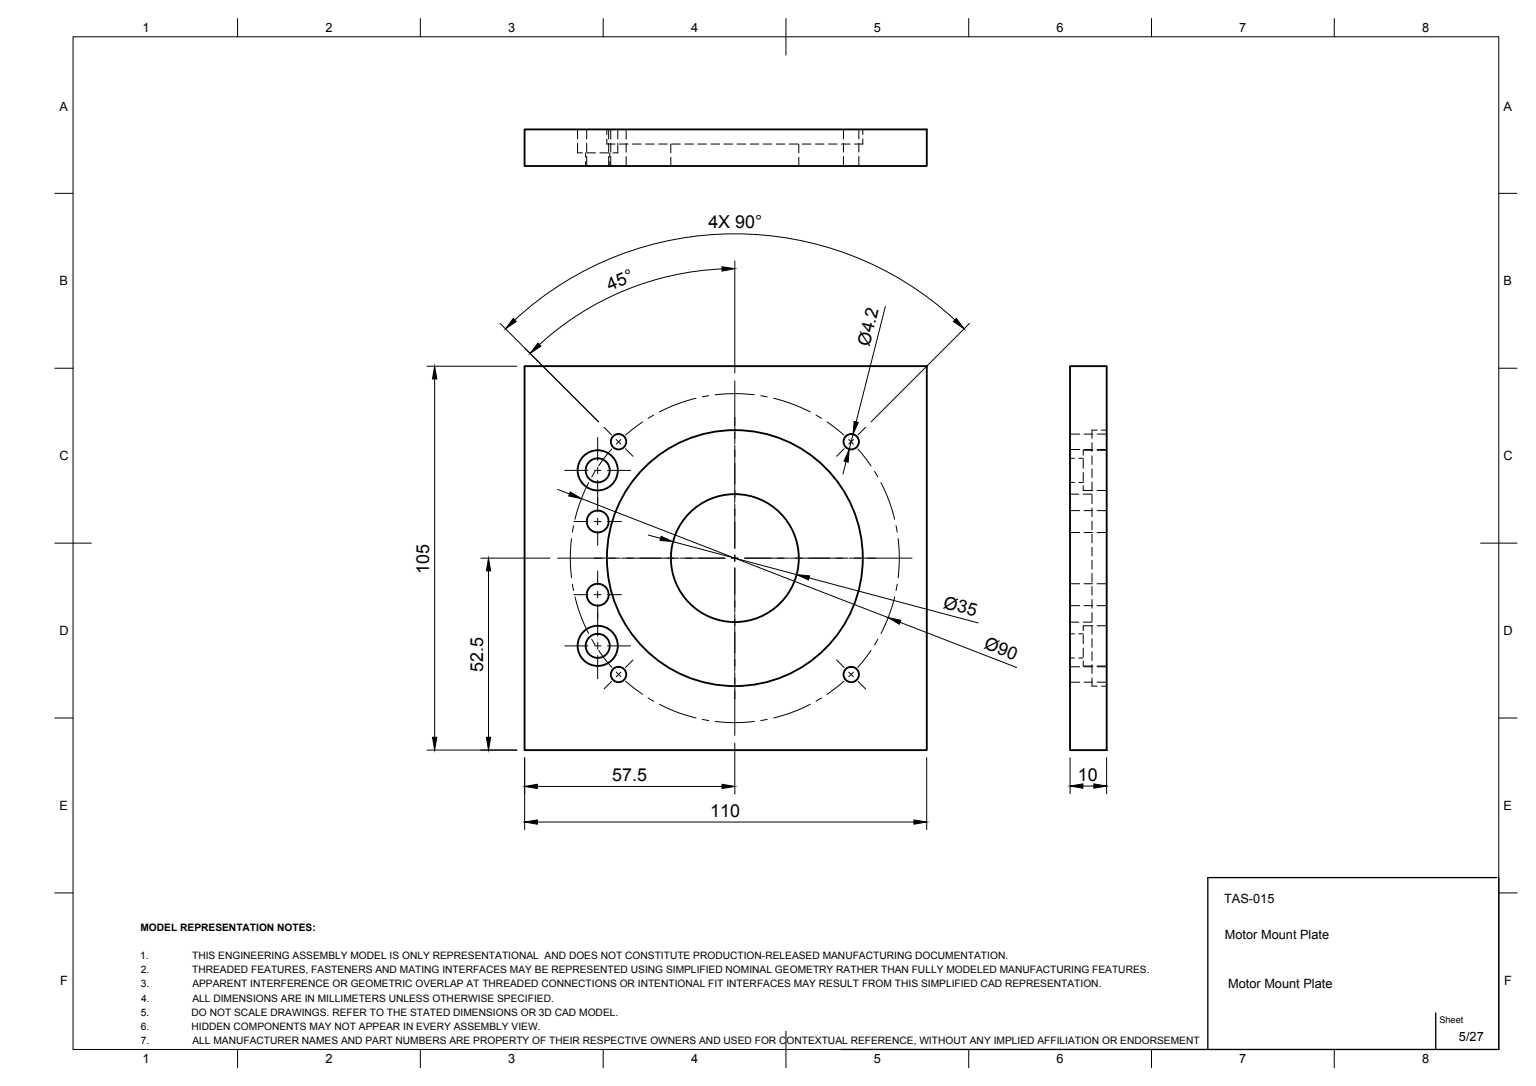
ISO-10303-21;
HEADER;
/* Generated by software containing ST-Developer
 * from STEP Tools, Inc. (www.steptools.com) 
 */

FILE_DESCRIPTION(
/* description */ ('STEP AP214'),
/* implementation_level */ '2;1');

FILE_NAME(
/* name */ 'Motor Mount Plate.step',
/* time_stamp */ '2026-11-15T14:49:54-08:00',
/* author */ (''),
/* organization */ (''),
/* preprocessor_version */ 'ST-DEVELOPER v20.2',
/* originating_system */ 'Autodesk Translation Framework v15.17.0.0',
/* authorisation */ '');

FILE_SCHEMA (('AUTOMOTIVE_DESIGN { 1 0 10303 214 3 1 1 }'));
ENDSEC;

DATA;
#10=MECHANICAL_DESIGN_GEOMETRIC_PRESENTATION_REPRESENTATION('',(#1100),#66721);
#1038=SHAPE_REPRESENTATION_RELATIONSHIP('SRR','None',#66894,#1069);
#1069=ADVANCED_BREP_SHAPE_REPRESENTATION('',(#1135),#66685);
#1100=STYLED_ITEM('',(#67095),#1135);
#1135=MANIFOLD_SOLID_BREP('Body1',#25666);
#1188=FACE_BOUND('',#3778,.T.);
#1189=FACE_BOUND('',#3779,.T.);
#1190=FACE_BOUND('',#3780,.T.);
#1191=FACE_BOUND('',#3781,.T.);
#1192=FACE_BOUND('',#3782,.T.);
#1193=FACE_BOUND('',#3783,.T.);
#1194=FACE_BOUND('',#3784,.T.);
#1195=FACE_BOUND('',#3785,.T.);
#1196=FACE_BOUND('',#3786,.T.);
#1197=FACE_BOUND('',#3792,.T.);
#1198=FACE_BOUND('',#3793,.T.);
#1199=FACE_BOUND('',#3794,.T.);
#1200=FACE_BOUND('',#3795,.T.);
#1201=FACE_BOUND('',#3796,.T.);
#1202=FACE_BOUND('',#3797,.T.);
#1203=FACE_BOUND('',#3798,.T.);
#1204=FACE_BOUND('',#3799,.T.);
#1205=FACE_BOUND('',#3800,.T.);
#1206=FACE_BOUND('',#3802,.T.);
#1207=FACE_BOUND('',#3804,.T.);
#1208=FACE_BOUND('',#3806,.T.);
#1524=PLANE('',#26132);
#1525=PLANE('',#26133);
#1526=PLANE('',#26134);
#1527=PLANE('',#26135);
#1528=PLANE('',#26136);
#1529=PLANE('',#26137);
#1530=PLANE('',#26138);
#1531=PLANE('',#26139);
#1532=PLANE('',#26140);
#2303=FACE_OUTER_BOUND('',#3765,.T.);
#2304=FACE_OUTER_BOUND('',#3766,.T.);
#2305=FACE_OUTER_BOUND('',#3767,.T.);
#2306=FACE_OUTER_BOUND('',#3768,.T.);
#2307=FACE_OUTER_BOUND('',#3769,.T.);
#2308=FACE_OUTER_BOUND('',#3770,.T.);
#2309=FACE_OUTER_BOUND('',#3771,.T.);
#2310=FACE_OUTER_BOUND('',#3772,.T.);
#2311=FACE_OUTER_BOUND('',#3773,.T.);
#2312=FACE_OUTER_BOUND('',#3774,.T.);
#2313=FACE_OUTER_BOUND('',#3775,.T.);
#2314=FACE_OUTER_BOUND('',#3776,.T.);
#2315=FACE_OUTER_BOUND('',#3777,.T.);
#2316=FACE_OUTER_BOUND('',#3787,.T.);
#2317=FACE_OUTER_BOUND('',#3788,.T.);
#2318=FACE_OUTER_BOUND('',#3789,.T.);
#2319=FACE_OUTER_BOUND('',#3790,.T.);
#2320=FACE_OUTER_BOUND('',#3791,.T.);
#2321=FACE_OUTER_BOUND('',#3801,.T.);
#2322=FACE_OUTER_BOUND('',#3803,.T.);
#2323=FACE_OUTER_BOUND('',#3805,.T.);
#3765=EDGE_LOOP('',(#16774,#16775,#16776,#16777));
#3766=EDGE_LOOP('',(#16778,#16779,#16780,#16781));
#3767=EDGE_LOOP('',(#16782,#16783,#16784,#16785));
#3768=EDGE_LOOP('',(#16786,#16787,#16788,#16789));
#3769=EDGE_LOOP('',(#16790,#16791,#16792,#16793));
#3770=EDGE_LOOP('',(#16794,#16795,#16796,#16797));
#3771=EDGE_LOOP('',(#16798,#16799,#16800,#16801));
#3772=EDGE_LOOP('',(#16802,#16803,#16804,#16805));
#3773=EDGE_LOOP('',(#16806,#16807,#16808,#16809));
#3774=EDGE_LOOP('',(#16810,#16811,#16812,#16813));
#3775=EDGE_LOOP('',(#16814,#16815,#16816,#16817));
#3776=EDGE_LOOP('',(#16818,#16819,#16820,#16821));
#3777=EDGE_LOOP('',(#16822,#16823,#16824,#16825));
#3778=EDGE_LOOP('',(#16826));
#3779=EDGE_LOOP('',(#16827));
#3780=EDGE_LOOP('',(#16828));
#3781=EDGE_LOOP('',(#16829));
#3782=EDGE_LOOP('',(#16830));
#3783=EDGE_LOOP('',(#16831));
#3784=EDGE_LOOP('',(#16832));
#3785=EDGE_LOOP('',(#16833));
#3786=EDGE_LOOP('',(#16834));
#3787=EDGE_LOOP('',(#16835,#16836,#16837,#16838));
#3788=EDGE_LOOP('',(#16839,#16840,#16841,#16842));
#3789=EDGE_LOOP('',(#16843,#16844,#16845,#16846));
#3790=EDGE_LOOP('',(#16847,#16848,#16849,#16850));
#3791=EDGE_LOOP('',(#16851,#16852,#16853,#16854));
#3792=EDGE_LOOP('',(#16855));
#3793=EDGE_LOOP('',(#16856));
#3794=EDGE_LOOP('',(#16857));
#3795=EDGE_LOOP('',(#16858));
#3796=EDGE_LOOP('',(#16859));
#3797=EDGE_LOOP('',(#16860));
#3798=EDGE_LOOP('',(#16861));
#3799=EDGE_LOOP('',(#16862));
#3800=EDGE_LOOP('',(#16863));
#3801=EDGE_LOOP('',(#16864));
#3802=EDGE_LOOP('',(#16865));
#3803=EDGE_LOOP('',(#16866));
#3804=EDGE_LOOP('',(#16867));
#3805=EDGE_LOOP('',(#16868));
#3806=EDGE_LOOP('',(#16869));
#5557=LINE('',#36368,#7546);
#5558=LINE('',#36374,#7547);
#5559=LINE('',#36380,#7548);
#5560=LINE('',#36386,#7549);
#5561=LINE('',#36392,#7550);
#5562=LINE('',#36398,#7551);
#5563=LINE('',#36404,#7552);
#5564=LINE('',#36410,#7553);
#5565=LINE('',#36416,#7554);
#5566=LINE('',#36422,#7555);
#5567=LINE('',#36428,#7556);
#5568=LINE('',#36434,#7557);
#5569=LINE('',#36439,#7558);
#5570=LINE('',#36441,#7559);
#5571=LINE('',#36443,#7560);
#5572=LINE('',#36444,#7561);
#5573=LINE('',#36447,#7562);
#5574=LINE('',#36449,#7563);
#5575=LINE('',#36450,#7564);
#5576=LINE('',#36453,#7565);
#5577=LINE('',#36454,#7566);
#5578=LINE('',#36457,#7567);
#5579=LINE('',#36458,#7568);
#5580=LINE('',#36460,#7569);
#7546=VECTOR('',#28944,2.1);
#7547=VECTOR('',#28951,2.1);
#7548=VECTOR('',#28958,2.1);
#7549=VECTOR('',#28965,2.1);
#7550=VECTOR('',#28972,3.);
#7551=VECTOR('',#28979,3.);
#7552=VECTOR('',#28986,5.5);
#7553=VECTOR('',#28993,3.3);
#7554=VECTOR('',#29000,5.5);
#7555=VECTOR('',#29007,3.3);
#7556=VECTOR('',#29014,17.5);
#7557=VECTOR('',#29021,35.);
#7558=VECTOR('',#29026,1000.);
#7559=VECTOR('',#29027,1000.);
#7560=VECTOR('',#29028,1000.);
#7561=VECTOR('',#29029,1000.);
#7562=VECTOR('',#29032,1000.);
#7563=VECTOR('',#29033,1000.);
#7564=VECTOR('',#29034,1000.);
#7565=VECTOR('',#29037,1000.);
#7566=VECTOR('',#29038,1000.);
#7567=VECTOR('',#29041,1000.);
#7568=VECTOR('',#29042,1000.);
#7569=VECTOR('',#29045,1000.);
#9477=CIRCLE('',#26097,2.1);
#9478=CIRCLE('',#26098,2.1);
#9479=CIRCLE('',#26100,2.1);
#9480=CIRCLE('',#26101,2.1);
#9481=CIRCLE('',#26103,2.1);
#9482=CIRCLE('',#26104,2.1);
#9483=CIRCLE('',#26106,2.1);
#9484=CIRCLE('',#26107,2.1);
#9485=CIRCLE('',#26109,3.);
#9486=CIRCLE('',#26110,3.);
#9487=CIRCLE('',#26112,3.);
#9488=CIRCLE('',#26113,3.);
#9489=CIRCLE('',#26115,5.5);
#9490=CIRCLE('',#26116,5.5);
#9491=CIRCLE('',#26118,3.3);
#9492=CIRCLE('',#26119,3.3);
#9493=CIRCLE('',#26121,5.5);
#9494=CIRCLE('',#26122,5.5);
#9495=CIRCLE('',#26124,3.3);
#9496=CIRCLE('',#26125,3.3);
#9497=CIRCLE('',#26127,17.5);
#9498=CIRCLE('',#26128,17.5);
#9499=CIRCLE('',#26130,35.);
#9500=CIRCLE('',#26131,35.);
#10698=VERTEX_POINT('',#36365);
#10699=VERTEX_POINT('',#36367);
#10700=VERTEX_POINT('',#36371);
#10701=VERTEX_POINT('',#36373);
#10702=VERTEX_POINT('',#36377);
#10703=VERTEX_POINT('',#36379);
#10704=VERTEX_POINT('',#36383);
#10705=VERTEX_POINT('',#36385);
#10706=VERTEX_POINT('',#36389);
#10707=VERTEX_POINT('',#36391);
#10708=VERTEX_POINT('',#36395);
#10709=VERTEX_POINT('',#36397);
#10710=VERTEX_POINT('',#36401);
#10711=VERTEX_POINT('',#36403);
#10712=VERTEX_POINT('',#36407);
#10713=VERTEX_POINT('',#36409);
#10714=VERTEX_POINT('',#36413);
#10715=VERTEX_POINT('',#36415);
#10716=VERTEX_POINT('',#36419);
#10717=VERTEX_POINT('',#36421);
#10718=VERTEX_POINT('',#36425);
#10719=VERTEX_POINT('',#36427);
#10720=VERTEX_POINT('',#36431);
#10721=VERTEX_POINT('',#36433);
#10722=VERTEX_POINT('',#36437);
#10723=VERTEX_POINT('',#36438);
#10724=VERTEX_POINT('',#36440);
#10725=VERTEX_POINT('',#36442);
#10726=VERTEX_POINT('',#36446);
#10727=VERTEX_POINT('',#36448);
#10728=VERTEX_POINT('',#36452);
#10729=VERTEX_POINT('',#36456);
#13080=EDGE_CURVE('',#10698,#10698,#9477,.T.);
#13081=EDGE_CURVE('',#10698,#10699,#5557,.T.);
#13082=EDGE_CURVE('',#10699,#10699,#9478,.T.);
#13083=EDGE_CURVE('',#10700,#10700,#9479,.T.);
#13084=EDGE_CURVE('',#10700,#10701,#5558,.T.);
#13085=EDGE_CURVE('',#10701,#10701,#9480,.T.);
#13086=EDGE_CURVE('',#10702,#10702,#9481,.T.);
#13087=EDGE_CURVE('',#10702,#10703,#5559,.T.);
#13088=EDGE_CURVE('',#10703,#10703,#9482,.T.);
#13089=EDGE_CURVE('',#10704,#10704,#9483,.T.);
#13090=EDGE_CURVE('',#10704,#10705,#5560,.T.);
#13091=EDGE_CURVE('',#10705,#10705,#9484,.T.);
#13092=EDGE_CURVE('',#10706,#10706,#9485,.T.);
#13093=EDGE_CURVE('',#10706,#10707,#5561,.T.);
#13094=EDGE_CURVE('',#10707,#10707,#9486,.T.);
#13095=EDGE_CURVE('',#10708,#10708,#9487,.T.);
#13096=EDGE_CURVE('',#10708,#10709,#5562,.T.);
#13097=EDGE_CURVE('',#10709,#10709,#9488,.T.);
#13098=EDGE_CURVE('',#10710,#10710,#9489,.T.);
#13099=EDGE_CURVE('',#10710,#10711,#5563,.T.);
#13100=EDGE_CURVE('',#10711,#10711,#9490,.T.);
#13101=EDGE_CURVE('',#10712,#10712,#9491,.T.);
#13102=EDGE_CURVE('',#10712,#10713,#5564,.T.);
#13103=EDGE_CURVE('',#10713,#10713,#9492,.T.);
#13104=EDGE_CURVE('',#10714,#10714,#9493,.T.);
#13105=EDGE_CURVE('',#10714,#10715,#5565,.T.);
#13106=EDGE_CURVE('',#10715,#10715,#9494,.T.);
#13107=EDGE_CURVE('',#10716,#10716,#9495,.T.);
#13108=EDGE_CURVE('',#10716,#10717,#5566,.T.);
#13109=EDGE_CURVE('',#10717,#10717,#9496,.T.);
#13110=EDGE_CURVE('',#10718,#10718,#9497,.T.);
#13111=EDGE_CURVE('',#10718,#10719,#5567,.T.);
#13112=EDGE_CURVE('',#10719,#10719,#9498,.T.);
#13113=EDGE_CURVE('',#10720,#10720,#9499,.T.);
#13114=EDGE_CURVE('',#10720,#10721,#5568,.T.);
#13115=EDGE_CURVE('',#10721,#10721,#9500,.T.);
#13116=EDGE_CURVE('',#10722,#10723,#5569,.T.);
#13117=EDGE_CURVE('',#10724,#10722,#5570,.T.);
#13118=EDGE_CURVE('',#10725,#10724,#5571,.T.);
#13119=EDGE_CURVE('',#10723,#10725,#5572,.T.);
#13120=EDGE_CURVE('',#10726,#10723,#5573,.T.);
#13121=EDGE_CURVE('',#10727,#10726,#5574,.T.);
#13122=EDGE_CURVE('',#10727,#10722,#5575,.T.);
#13123=EDGE_CURVE('',#10728,#10725,#5576,.T.);
#13124=EDGE_CURVE('',#10726,#10728,#5577,.T.);
#13125=EDGE_CURVE('',#10729,#10724,#5578,.T.);
#13126=EDGE_CURVE('',#10728,#10729,#5579,.T.);
#13127=EDGE_CURVE('',#10729,#10727,#5580,.T.);
#16774=ORIENTED_EDGE('',*,*,#13080,.F.);
#16775=ORIENTED_EDGE('',*,*,#13081,.T.);
#16776=ORIENTED_EDGE('',*,*,#13082,.T.);
#16777=ORIENTED_EDGE('',*,*,#13081,.F.);
#16778=ORIENTED_EDGE('',*,*,#13083,.F.);
#16779=ORIENTED_EDGE('',*,*,#13084,.T.);
#16780=ORIENTED_EDGE('',*,*,#13085,.T.);
#16781=ORIENTED_EDGE('',*,*,#13084,.F.);
#16782=ORIENTED_EDGE('',*,*,#13086,.F.);
#16783=ORIENTED_EDGE('',*,*,#13087,.T.);
#16784=ORIENTED_EDGE('',*,*,#13088,.T.);
#16785=ORIENTED_EDGE('',*,*,#13087,.F.);
#16786=ORIENTED_EDGE('',*,*,#13089,.F.);
#16787=ORIENTED_EDGE('',*,*,#13090,.T.);
#16788=ORIENTED_EDGE('',*,*,#13091,.T.);
#16789=ORIENTED_EDGE('',*,*,#13090,.F.);
#16790=ORIENTED_EDGE('',*,*,#13092,.F.);
#16791=ORIENTED_EDGE('',*,*,#13093,.T.);
#16792=ORIENTED_EDGE('',*,*,#13094,.T.);
#16793=ORIENTED_EDGE('',*,*,#13093,.F.);
#16794=ORIENTED_EDGE('',*,*,#13095,.F.);
#16795=ORIENTED_EDGE('',*,*,#13096,.T.);
#16796=ORIENTED_EDGE('',*,*,#13097,.T.);
#16797=ORIENTED_EDGE('',*,*,#13096,.F.);
#16798=ORIENTED_EDGE('',*,*,#13098,.F.);
#16799=ORIENTED_EDGE('',*,*,#13099,.T.);
#16800=ORIENTED_EDGE('',*,*,#13100,.T.);
#16801=ORIENTED_EDGE('',*,*,#13099,.F.);
#16802=ORIENTED_EDGE('',*,*,#13101,.F.);
#16803=ORIENTED_EDGE('',*,*,#13102,.T.);
#16804=ORIENTED_EDGE('',*,*,#13103,.T.);
#16805=ORIENTED_EDGE('',*,*,#13102,.F.);
#16806=ORIENTED_EDGE('',*,*,#13104,.F.);
#16807=ORIENTED_EDGE('',*,*,#13105,.T.);
#16808=ORIENTED_EDGE('',*,*,#13106,.T.);
#16809=ORIENTED_EDGE('',*,*,#13105,.F.);
#16810=ORIENTED_EDGE('',*,*,#13107,.F.);
#16811=ORIENTED_EDGE('',*,*,#13108,.T.);
#16812=ORIENTED_EDGE('',*,*,#13109,.T.);
#16813=ORIENTED_EDGE('',*,*,#13108,.F.);
#16814=ORIENTED_EDGE('',*,*,#13110,.F.);
#16815=ORIENTED_EDGE('',*,*,#13111,.T.);
#16816=ORIENTED_EDGE('',*,*,#13112,.T.);
#16817=ORIENTED_EDGE('',*,*,#13111,.F.);
#16818=ORIENTED_EDGE('',*,*,#13113,.F.);
#16819=ORIENTED_EDGE('',*,*,#13114,.T.);
#16820=ORIENTED_EDGE('',*,*,#13115,.T.);
#16821=ORIENTED_EDGE('',*,*,#13114,.F.);
#16822=ORIENTED_EDGE('',*,*,#13116,.F.);
#16823=ORIENTED_EDGE('',*,*,#13117,.F.);
#16824=ORIENTED_EDGE('',*,*,#13118,.F.);
#16825=ORIENTED_EDGE('',*,*,#13119,.F.);
#16826=ORIENTED_EDGE('',*,*,#13110,.T.);
#16827=ORIENTED_EDGE('',*,*,#13107,.T.);
#16828=ORIENTED_EDGE('',*,*,#13101,.T.);
#16829=ORIENTED_EDGE('',*,*,#13095,.T.);
#16830=ORIENTED_EDGE('',*,*,#13092,.T.);
#16831=ORIENTED_EDGE('',*,*,#13089,.T.);
#16832=ORIENTED_EDGE('',*,*,#13086,.T.);
#16833=ORIENTED_EDGE('',*,*,#13080,.T.);
#16834=ORIENTED_EDGE('',*,*,#13083,.T.);
#16835=ORIENTED_EDGE('',*,*,#13116,.T.);
#16836=ORIENTED_EDGE('',*,*,#13120,.F.);
#16837=ORIENTED_EDGE('',*,*,#13121,.F.);
#16838=ORIENTED_EDGE('',*,*,#13122,.T.);
#16839=ORIENTED_EDGE('',*,*,#13119,.T.);
#16840=ORIENTED_EDGE('',*,*,#13123,.F.);
#16841=ORIENTED_EDGE('',*,*,#13124,.F.);
#16842=ORIENTED_EDGE('',*,*,#13120,.T.);
#16843=ORIENTED_EDGE('',*,*,#13118,.T.);
#16844=ORIENTED_EDGE('',*,*,#13125,.F.);
#16845=ORIENTED_EDGE('',*,*,#13126,.F.);
#16846=ORIENTED_EDGE('',*,*,#13123,.T.);
#16847=ORIENTED_EDGE('',*,*,#13117,.T.);
#16848=ORIENTED_EDGE('',*,*,#13122,.F.);
#16849=ORIENTED_EDGE('',*,*,#13127,.F.);
#16850=ORIENTED_EDGE('',*,*,#13125,.T.);
#16851=ORIENTED_EDGE('',*,*,#13121,.T.);
#16852=ORIENTED_EDGE('',*,*,#13124,.T.);
#16853=ORIENTED_EDGE('',*,*,#13126,.T.);
#16854=ORIENTED_EDGE('',*,*,#13127,.T.);
#16855=ORIENTED_EDGE('',*,*,#13082,.F.);
#16856=ORIENTED_EDGE('',*,*,#13085,.F.);
#16857=ORIENTED_EDGE('',*,*,#13088,.F.);
#16858=ORIENTED_EDGE('',*,*,#13091,.F.);
#16859=ORIENTED_EDGE('',*,*,#13094,.F.);
#16860=ORIENTED_EDGE('',*,*,#13097,.F.);
#16861=ORIENTED_EDGE('',*,*,#13100,.F.);
#16862=ORIENTED_EDGE('',*,*,#13106,.F.);
#16863=ORIENTED_EDGE('',*,*,#13115,.F.);
#16864=ORIENTED_EDGE('',*,*,#13113,.T.);
#16865=ORIENTED_EDGE('',*,*,#13112,.F.);
#16866=ORIENTED_EDGE('',*,*,#13104,.T.);
#16867=ORIENTED_EDGE('',*,*,#13109,.F.);
#16868=ORIENTED_EDGE('',*,*,#13098,.T.);
#16869=ORIENTED_EDGE('',*,*,#13103,.F.);
#23810=CYLINDRICAL_SURFACE('',#26096,2.1);
#23811=CYLINDRICAL_SURFACE('',#26099,2.1);
#23812=CYLINDRICAL_SURFACE('',#26102,2.1);
#23813=CYLINDRICAL_SURFACE('',#26105,2.1);
#23814=CYLINDRICAL_SURFACE('',#26108,3.);
#23815=CYLINDRICAL_SURFACE('',#26111,3.);
#23816=CYLINDRICAL_SURFACE('',#26114,5.5);
#23817=CYLINDRICAL_SURFACE('',#26117,3.3);
#23818=CYLINDRICAL_SURFACE('',#26120,5.5);
#23819=CYLINDRICAL_SURFACE('',#26123,3.3);
#23820=CYLINDRICAL_SURFACE('',#26126,17.5);
#23821=CYLINDRICAL_SURFACE('',#26129,35.);
#24256=ADVANCED_FACE('',(#2303),#23810,.F.);
#24257=ADVANCED_FACE('',(#2304),#23811,.F.);
#24258=ADVANCED_FACE('',(#2305),#23812,.F.);
#24259=ADVANCED_FACE('',(#2306),#23813,.F.);
#24260=ADVANCED_FACE('',(#2307),#23814,.F.);
#24261=ADVANCED_FACE('',(#2308),#23815,.F.);
#24262=ADVANCED_FACE('',(#2309),#23816,.F.);
#24263=ADVANCED_FACE('',(#2310),#23817,.F.);
#24264=ADVANCED_FACE('',(#2311),#23818,.F.);
#24265=ADVANCED_FACE('',(#2312),#23819,.F.);
#24266=ADVANCED_FACE('',(#2313),#23820,.F.);
#24267=ADVANCED_FACE('',(#2314),#23821,.F.);
#24268=ADVANCED_FACE('',(#2315,#1188,#1189,#1190,#1191,#1192,#1193,#1194,
#1195,#1196),#1524,.T.);
#24269=ADVANCED_FACE('',(#2316),#1525,.F.);
#24270=ADVANCED_FACE('',(#2317),#1526,.F.);
#24271=ADVANCED_FACE('',(#2318),#1527,.F.);
#24272=ADVANCED_FACE('',(#2319),#1528,.F.);
#24273=ADVANCED_FACE('',(#2320,#1197,#1198,#1199,#1200,#1201,#1202,#1203,
#1204,#1205),#1529,.F.);
#24274=ADVANCED_FACE('',(#2321,#1206),#1530,.T.);
#24275=ADVANCED_FACE('',(#2322,#1207),#1531,.F.);
#24276=ADVANCED_FACE('',(#2323,#1208),#1532,.F.);
#25666=CLOSED_SHELL('',(#24256,#24257,#24258,#24259,#24260,#24261,#24262,
#24263,#24264,#24265,#24266,#24267,#24268,#24269,#24270,#24271,#24272,#24273,
#24274,#24275,#24276));
#26095=AXIS2_PLACEMENT_3D('',#36363,#28938,#28939);
#26096=AXIS2_PLACEMENT_3D('',#36364,#28940,#28941);
#26097=AXIS2_PLACEMENT_3D('',#36366,#28942,#28943);
#26098=AXIS2_PLACEMENT_3D('',#36369,#28945,#28946);
#26099=AXIS2_PLACEMENT_3D('',#36370,#28947,#28948);
#26100=AXIS2_PLACEMENT_3D('',#36372,#28949,#28950);
#26101=AXIS2_PLACEMENT_3D('',#36375,#28952,#28953);
#26102=AXIS2_PLACEMENT_3D('',#36376,#28954,#28955);
#26103=AXIS2_PLACEMENT_3D('',#36378,#28956,#28957);
#26104=AXIS2_PLACEMENT_3D('',#36381,#28959,#28960);
#26105=AXIS2_PLACEMENT_3D('',#36382,#28961,#28962);
#26106=AXIS2_PLACEMENT_3D('',#36384,#28963,#28964);
#26107=AXIS2_PLACEMENT_3D('',#36387,#28966,#28967);
#26108=AXIS2_PLACEMENT_3D('',#36388,#28968,#28969);
#26109=AXIS2_PLACEMENT_3D('',#36390,#28970,#28971);
#26110=AXIS2_PLACEMENT_3D('',#36393,#28973,#28974);
#26111=AXIS2_PLACEMENT_3D('',#36394,#28975,#28976);
#26112=AXIS2_PLACEMENT_3D('',#36396,#28977,#28978);
#26113=AXIS2_PLACEMENT_3D('',#36399,#28980,#28981);
#26114=AXIS2_PLACEMENT_3D('',#36400,#28982,#28983);
#26115=AXIS2_PLACEMENT_3D('',#36402,#28984,#28985);
#26116=AXIS2_PLACEMENT_3D('',#36405,#28987,#28988);
#26117=AXIS2_PLACEMENT_3D('',#36406,#28989,#28990);
#26118=AXIS2_PLACEMENT_3D('',#36408,#28991,#28992);
#26119=AXIS2_PLACEMENT_3D('',#36411,#28994,#28995);
#26120=AXIS2_PLACEMENT_3D('',#36412,#28996,#28997);
#26121=AXIS2_PLACEMENT_3D('',#36414,#28998,#28999);
#26122=AXIS2_PLACEMENT_3D('',#36417,#29001,#29002);
#26123=AXIS2_PLACEMENT_3D('',#36418,#29003,#29004);
#26124=AXIS2_PLACEMENT_3D('',#36420,#29005,#29006);
#26125=AXIS2_PLACEMENT_3D('',#36423,#29008,#29009);
#26126=AXIS2_PLACEMENT_3D('',#36424,#29010,#29011);
#26127=AXIS2_PLACEMENT_3D('',#36426,#29012,#29013);
#26128=AXIS2_PLACEMENT_3D('',#36429,#29015,#29016);
#26129=AXIS2_PLACEMENT_3D('',#36430,#29017,#29018);
#26130=AXIS2_PLACEMENT_3D('',#36432,#29019,#29020);
#26131=AXIS2_PLACEMENT_3D('',#36435,#29022,#29023);
#26132=AXIS2_PLACEMENT_3D('',#36436,#29024,#29025);
#26133=AXIS2_PLACEMENT_3D('',#36445,#29030,#29031);
#26134=AXIS2_PLACEMENT_3D('',#36451,#29035,#29036);
#26135=AXIS2_PLACEMENT_3D('',#36455,#29039,#29040);
#26136=AXIS2_PLACEMENT_3D('',#36459,#29043,#29044);
#26137=AXIS2_PLACEMENT_3D('',#36461,#29046,#29047);
#26138=AXIS2_PLACEMENT_3D('',#36462,#29048,#29049);
#26139=AXIS2_PLACEMENT_3D('',#36463,#29050,#29051);
#26140=AXIS2_PLACEMENT_3D('',#36464,#29052,#29053);
#28938=DIRECTION('axis',(0.,0.,1.));
#28939=DIRECTION('refdir',(1.,0.,0.));
#28940=DIRECTION('center_axis',(0.,0.,1.));
#28941=DIRECTION('ref_axis',(1.,0.,0.));
#28942=DIRECTION('center_axis',(0.,0.,1.));
#28943=DIRECTION('ref_axis',(1.,0.,0.));
#28944=DIRECTION('',(0.,0.,1.));
#28945=DIRECTION('center_axis',(0.,0.,1.));
#28946=DIRECTION('ref_axis',(1.,0.,0.));
#28947=DIRECTION('center_axis',(0.,0.,1.));
#28948=DIRECTION('ref_axis',(1.,0.,0.));
#28949=DIRECTION('center_axis',(0.,0.,1.));
#28950=DIRECTION('ref_axis',(1.,0.,0.));
#28951=DIRECTION('',(0.,0.,1.));
#28952=DIRECTION('center_axis',(0.,0.,1.));
#28953=DIRECTION('ref_axis',(1.,0.,0.));
#28954=DIRECTION('center_axis',(0.,0.,1.));
#28955=DIRECTION('ref_axis',(1.,0.,0.));
#28956=DIRECTION('center_axis',(0.,0.,1.));
#28957=DIRECTION('ref_axis',(1.,0.,0.));
#28958=DIRECTION('',(0.,0.,1.));
#28959=DIRECTION('center_axis',(0.,0.,1.));
#28960=DIRECTION('ref_axis',(1.,0.,0.));
#28961=DIRECTION('center_axis',(0.,0.,1.));
#28962=DIRECTION('ref_axis',(1.,0.,0.));
#28963=DIRECTION('center_axis',(0.,0.,1.));
#28964=DIRECTION('ref_axis',(1.,0.,0.));
#28965=DIRECTION('',(0.,0.,1.));
#28966=DIRECTION('center_axis',(0.,0.,1.));
#28967=DIRECTION('ref_axis',(1.,0.,0.));
#28968=DIRECTION('center_axis',(0.,0.,1.));
#28969=DIRECTION('ref_axis',(1.,0.,0.));
#28970=DIRECTION('center_axis',(0.,0.,1.));
#28971=DIRECTION('ref_axis',(1.,0.,0.));
#28972=DIRECTION('',(0.,0.,1.));
#28973=DIRECTION('center_axis',(0.,0.,1.));
#28974=DIRECTION('ref_axis',(1.,0.,0.));
#28975=DIRECTION('center_axis',(0.,0.,1.));
#28976=DIRECTION('ref_axis',(1.,0.,0.));
#28977=DIRECTION('center_axis',(0.,0.,1.));
#28978=DIRECTION('ref_axis',(1.,0.,0.));
#28979=DIRECTION('',(0.,0.,1.));
#28980=DIRECTION('center_axis',(0.,0.,1.));
#28981=DIRECTION('ref_axis',(1.,0.,0.));
#28982=DIRECTION('center_axis',(0.,0.,1.));
#28983=DIRECTION('ref_axis',(1.,0.,0.));
#28984=DIRECTION('center_axis',(0.,0.,1.));
#28985=DIRECTION('ref_axis',(1.,0.,0.));
#28986=DIRECTION('',(0.,0.,1.));
#28987=DIRECTION('center_axis',(0.,0.,1.));
#28988=DIRECTION('ref_axis',(1.,0.,0.));
#28989=DIRECTION('center_axis',(0.,0.,1.));
#28990=DIRECTION('ref_axis',(1.,0.,0.));
#28991=DIRECTION('center_axis',(0.,0.,1.));
#28992=DIRECTION('ref_axis',(1.,0.,0.));
#28993=DIRECTION('',(0.,0.,1.));
#28994=DIRECTION('center_axis',(0.,0.,1.));
#28995=DIRECTION('ref_axis',(1.,0.,0.));
#28996=DIRECTION('center_axis',(0.,0.,1.));
#28997=DIRECTION('ref_axis',(1.,0.,0.));
#28998=DIRECTION('center_axis',(0.,0.,1.));
#28999=DIRECTION('ref_axis',(1.,0.,0.));
#29000=DIRECTION('',(0.,0.,1.));
#29001=DIRECTION('center_axis',(0.,0.,1.));
#29002=DIRECTION('ref_axis',(1.,0.,0.));
#29003=DIRECTION('center_axis',(0.,0.,1.));
#29004=DIRECTION('ref_axis',(1.,0.,0.));
#29005=DIRECTION('center_axis',(0.,0.,1.));
#29006=DIRECTION('ref_axis',(1.,0.,0.));
#29007=DIRECTION('',(0.,0.,1.));
#29008=DIRECTION('center_axis',(0.,0.,1.));
#29009=DIRECTION('ref_axis',(1.,0.,0.));
#29010=DIRECTION('center_axis',(0.,0.,1.));
#29011=DIRECTION('ref_axis',(1.,0.,0.));
#29012=DIRECTION('center_axis',(0.,0.,1.));
#29013=DIRECTION('ref_axis',(1.,0.,0.));
#29014=DIRECTION('',(0.,0.,1.));
#29015=DIRECTION('center_axis',(0.,0.,1.));
#29016=DIRECTION('ref_axis',(1.,0.,0.));
#29017=DIRECTION('center_axis',(0.,0.,1.));
#29018=DIRECTION('ref_axis',(1.,0.,0.));
#29019=DIRECTION('center_axis',(0.,0.,1.));
#29020=DIRECTION('ref_axis',(1.,0.,0.));
#29021=DIRECTION('',(0.,0.,1.));
#29022=DIRECTION('center_axis',(0.,0.,1.));
#29023=DIRECTION('ref_axis',(1.,0.,0.));
#29024=DIRECTION('center_axis',(0.,0.,-1.));
#29025=DIRECTION('ref_axis',(-1.,0.,0.));
#29026=DIRECTION('',(0.,1.,0.));
#29027=DIRECTION('',(1.,0.,0.));
#29028=DIRECTION('',(0.,-1.,0.));
#29029=DIRECTION('',(-1.,0.,0.));
#29030=DIRECTION('center_axis',(-1.,0.,0.));
#29031=DIRECTION('ref_axis',(0.,0.,1.));
#29032=DIRECTION('',(0.,0.,-1.));
#29033=DIRECTION('',(0.,1.,0.));
#29034=DIRECTION('',(0.,0.,-1.));
#29035=DIRECTION('center_axis',(0.,-1.,0.));
#29036=DIRECTION('ref_axis',(0.,0.,-1.));
#29037=DIRECTION('',(0.,0.,-1.));
#29038=DIRECTION('',(-1.,0.,0.));
#29039=DIRECTION('center_axis',(1.,0.,0.));
#29040=DIRECTION('ref_axis',(0.,0.,-1.));
#29041=DIRECTION('',(0.,0.,-1.));
#29042=DIRECTION('',(0.,-1.,0.));
#29043=DIRECTION('center_axis',(0.,1.,0.));
#29044=DIRECTION('ref_axis',(0.,0.,1.));
#29045=DIRECTION('',(1.,0.,0.));
#29046=DIRECTION('center_axis',(0.,0.,-1.));
#29047=DIRECTION('ref_axis',(-1.,0.,0.));
#29048=DIRECTION('center_axis',(0.,0.,1.));
#29049=DIRECTION('ref_axis',(1.,0.,0.));
#29050=DIRECTION('center_axis',(0.,0.,-1.));
#29051=DIRECTION('ref_axis',(-1.,0.,0.));
#29052=DIRECTION('center_axis',(0.,0.,-1.));
#29053=DIRECTION('ref_axis',(-1.,0.,0.));
#36363=CARTESIAN_POINT('',(0.,0.,0.));
#36364=CARTESIAN_POINT('Origin',(31.819805153395,29.3198051533945,5.));
#36365=CARTESIAN_POINT('',(29.719805153395,29.3198051533945,-5.));
#36366=CARTESIAN_POINT('Origin',(31.819805153395,29.3198051533945,-5.));
#36367=CARTESIAN_POINT('',(29.719805153395,29.3198051533945,5.));
#36368=CARTESIAN_POINT('',(29.719805153395,29.3198051533945,5.));
#36369=CARTESIAN_POINT('Origin',(31.819805153395,29.3198051533945,5.));
#36370=CARTESIAN_POINT('Origin',(-31.8198051533946,29.319805153395,5.));
#36371=CARTESIAN_POINT('',(-33.9198051533946,29.319805153395,-5.));
#36372=CARTESIAN_POINT('Origin',(-31.8198051533946,29.319805153395,-5.));
#36373=CARTESIAN_POINT('',(-33.9198051533946,29.319805153395,5.));
#36374=CARTESIAN_POINT('',(-33.9198051533946,29.319805153395,5.));
#36375=CARTESIAN_POINT('Origin',(-31.8198051533946,29.319805153395,5.));
#36376=CARTESIAN_POINT('Origin',(-31.8198051533948,-34.3198051533942,5.));
#36377=CARTESIAN_POINT('',(-33.9198051533948,-34.3198051533942,-5.));
#36378=CARTESIAN_POINT('Origin',(-31.8198051533948,-34.3198051533942,-5.));
#36379=CARTESIAN_POINT('',(-33.9198051533948,-34.3198051533942,5.));
#36380=CARTESIAN_POINT('',(-33.9198051533948,-34.3198051533942,5.));
#36381=CARTESIAN_POINT('Origin',(-31.8198051533948,-34.3198051533942,5.));
#36382=CARTESIAN_POINT('Origin',(31.8198051533946,-34.3198051533944,5.));
#36383=CARTESIAN_POINT('',(29.7198051533946,-34.3198051533944,-5.));
#36384=CARTESIAN_POINT('Origin',(31.8198051533946,-34.3198051533944,-5.));
#36385=CARTESIAN_POINT('',(29.7198051533946,-34.3198051533944,5.));
#36386=CARTESIAN_POINT('',(29.7198051533946,-34.3198051533944,5.));
#36387=CARTESIAN_POINT('Origin',(31.8198051533946,-34.3198051533944,5.));
#36388=CARTESIAN_POINT('Origin',(-10.,35.,5.));
#36389=CARTESIAN_POINT('',(-13.,35.,-5.));
#36390=CARTESIAN_POINT('Origin',(-10.,35.,-5.));
#36391=CARTESIAN_POINT('',(-13.,35.,5.));
#36392=CARTESIAN_POINT('',(-13.,35.,5.));
#36393=CARTESIAN_POINT('Origin',(-10.,35.,5.));
#36394=CARTESIAN_POINT('Origin',(10.,35.,5.));
#36395=CARTESIAN_POINT('',(7.,35.,-5.));
#36396=CARTESIAN_POINT('Origin',(10.,35.,-5.));
#36397=CARTESIAN_POINT('',(7.,35.,5.));
#36398=CARTESIAN_POINT('',(7.,35.,5.));
#36399=CARTESIAN_POINT('Origin',(10.,35.,5.));
#36400=CARTESIAN_POINT('Origin',(-24.,35.,5.));
#36401=CARTESIAN_POINT('',(-29.5,35.,-1.4));
#36402=CARTESIAN_POINT('Origin',(-24.,35.,-1.4));
#36403=CARTESIAN_POINT('',(-29.5,35.,5.));
#36404=CARTESIAN_POINT('',(-29.5,35.,5.));
#36405=CARTESIAN_POINT('Origin',(-24.,35.,5.));
#36406=CARTESIAN_POINT('Origin',(-24.,35.,5.));
#36407=CARTESIAN_POINT('',(-27.3,35.,-5.));
#36408=CARTESIAN_POINT('Origin',(-24.,35.,-5.));
#36409=CARTESIAN_POINT('',(-27.3,35.,-1.4));
#36410=CARTESIAN_POINT('',(-27.3,35.,5.));
#36411=CARTESIAN_POINT('Origin',(-24.,35.,-1.4));
#36412=CARTESIAN_POINT('Origin',(24.,35.,5.));
#36413=CARTESIAN_POINT('',(18.5,35.,-1.4));
#36414=CARTESIAN_POINT('Origin',(24.,35.,-1.4));
#36415=CARTESIAN_POINT('',(18.5,35.,5.));
#36416=CARTESIAN_POINT('',(18.5,35.,5.));
#36417=CARTESIAN_POINT('Origin',(24.,35.,5.));
#36418=CARTESIAN_POINT('Origin',(24.,35.,5.));
#36419=CARTESIAN_POINT('',(20.7,35.,-5.));
#36420=CARTESIAN_POINT('Origin',(24.,35.,-5.));
#36421=CARTESIAN_POINT('',(20.7,35.,-1.4));
#36422=CARTESIAN_POINT('',(20.7,35.,5.));
#36423=CARTESIAN_POINT('Origin',(24.,35.,-1.4));
#36424=CARTESIAN_POINT('Origin',(-1.20882209737476E-14,-2.49999999999972,
-5.));
#36425=CARTESIAN_POINT('',(-17.5,-2.49999999999972,-5.));
#36426=CARTESIAN_POINT('Origin',(-1.20882209737476E-14,-2.49999999999972,
-5.));
#36427=CARTESIAN_POINT('',(-17.5,-2.49999999999972,1.));
#36428=CARTESIAN_POINT('',(-17.5,-2.49999999999972,-5.));
#36429=CARTESIAN_POINT('Origin',(-1.20882209737476E-14,-2.49999999999972,
1.));
#36430=CARTESIAN_POINT('Origin',(-1.20882209737476E-14,-2.49999999999972,
1.));
#36431=CARTESIAN_POINT('',(-35.,-2.49999999999972,1.));
#36432=CARTESIAN_POINT('Origin',(-1.20882209737476E-14,-2.49999999999972,
1.));
#36433=CARTESIAN_POINT('',(-35.,-2.49999999999972,5.));
#36434=CARTESIAN_POINT('',(-35.,-2.49999999999972,1.));
#36435=CARTESIAN_POINT('Origin',(-1.20882209737476E-14,-2.49999999999972,
5.));
#36436=CARTESIAN_POINT('Origin',(0.,0.,-5.));
#36437=CARTESIAN_POINT('',(52.5,-55.,-5.));
#36438=CARTESIAN_POINT('',(52.5,55.,-5.));
#36439=CARTESIAN_POINT('',(52.5,-55.,-5.));
#36440=CARTESIAN_POINT('',(-52.5,-55.,-5.));
#36441=CARTESIAN_POINT('',(-52.5,-55.,-5.));
#36442=CARTESIAN_POINT('',(-52.5,55.,-5.));
#36443=CARTESIAN_POINT('',(-52.5,-55.,-5.));
#36444=CARTESIAN_POINT('',(-52.5,55.,-5.));
#36445=CARTESIAN_POINT('Origin',(52.5,-55.,5.));
#36446=CARTESIAN_POINT('',(52.5,55.,5.));
#36447=CARTESIAN_POINT('',(52.5,55.,5.));
#36448=CARTESIAN_POINT('',(52.5,-55.,5.));
#36449=CARTESIAN_POINT('',(52.5,-55.,5.));
#36450=CARTESIAN_POINT('',(52.5,-55.,5.));
#36451=CARTESIAN_POINT('Origin',(-52.5,55.,5.));
#36452=CARTESIAN_POINT('',(-52.5,55.,5.));
#36453=CARTESIAN_POINT('',(-52.5,55.,5.));
#36454=CARTESIAN_POINT('',(-52.5,55.,5.));
#36455=CARTESIAN_POINT('Origin',(-52.5,-55.,5.));
#36456=CARTESIAN_POINT('',(-52.5,-55.,5.));
#36457=CARTESIAN_POINT('',(-52.5,-55.,5.));
#36458=CARTESIAN_POINT('',(-52.5,-55.,5.));
#36459=CARTESIAN_POINT('Origin',(-52.5,-55.,5.));
#36460=CARTESIAN_POINT('',(-52.5,-55.,5.));
#36461=CARTESIAN_POINT('Origin',(0.,0.,5.));
#36462=CARTESIAN_POINT('Origin',(-1.20882209737476E-14,-2.49999999999972,
1.));
#36463=CARTESIAN_POINT('Origin',(27.3,35.,-1.4));
#36464=CARTESIAN_POINT('Origin',(-20.7,35.,-1.4));
#66644=UNCERTAINTY_MEASURE_WITH_UNIT(LENGTH_MEASURE(0.01),#66722,
'DISTANCE_ACCURACY_VALUE',
'Maximum model space distance between geometric entities at asserted c
onnectivities');
#66680=UNCERTAINTY_MEASURE_WITH_UNIT(LENGTH_MEASURE(0.01),#66722,
'DISTANCE_ACCURACY_VALUE',
'Maximum model space distance between geometric entities at asserted c
onnectivities');
#66685=(
GEOMETRIC_REPRESENTATION_CONTEXT(3)
GLOBAL_UNCERTAINTY_ASSIGNED_CONTEXT((#66644))
GLOBAL_UNIT_ASSIGNED_CONTEXT((#66722,#66724,#66725))
REPRESENTATION_CONTEXT('','3D')
);
#66721=(
GEOMETRIC_REPRESENTATION_CONTEXT(3)
GLOBAL_UNCERTAINTY_ASSIGNED_CONTEXT((#66680))
GLOBAL_UNIT_ASSIGNED_CONTEXT((#66722,#66724,#66725))
REPRESENTATION_CONTEXT('','3D')
);
#66722=(
LENGTH_UNIT()
NAMED_UNIT(*)
SI_UNIT(.MILLI.,.METRE.)
);
#66724=(
NAMED_UNIT(*)
PLANE_ANGLE_UNIT()
SI_UNIT($,.RADIAN.)
);
#66725=(
NAMED_UNIT(*)
SI_UNIT($,.STERADIAN.)
SOLID_ANGLE_UNIT()
);
#66730=SHAPE_DEFINITION_REPRESENTATION(#66770,#66894);
#66770=PRODUCT_DEFINITION_SHAPE('',$,#66935);
#66894=SHAPE_REPRESENTATION('',(#26095),#66685);
#66930=PRODUCT_DEFINITION_CONTEXT('part definition',#67052,'design');
#66935=PRODUCT_DEFINITION('Motor Mount Plate','Motor Mount Plate',#66975,
#66930);
#66975=PRODUCT_DEFINITION_FORMATION('',$,#67058);
#67052=APPLICATION_CONTEXT(
'Core Data for Automotive Mechanical Design Process');
#67053=PRODUCT_CONTEXT('part definition',#67052,'mechanical');
#67058=PRODUCT('Motor Mount Plate','Motor Mount Plate',$,(#67053));
#67095=PRESENTATION_STYLE_ASSIGNMENT((#67097));
#67097=SURFACE_STYLE_USAGE(.BOTH.,#67099);
#67099=SURFACE_SIDE_STYLE('',(#67101));
#67101=SURFACE_STYLE_FILL_AREA(#67103);
#67103=FILL_AREA_STYLE('Opaque(202,209,238)',(#67105));
#67105=FILL_AREA_STYLE_COLOUR('Opaque(202,209,238)',#67107);
#67107=COLOUR_RGB('Opaque(202,209,238)',0.792156862745098,0.819607843137255,
0.933333333333333);
ENDSEC;
END-ISO-10303-21;
